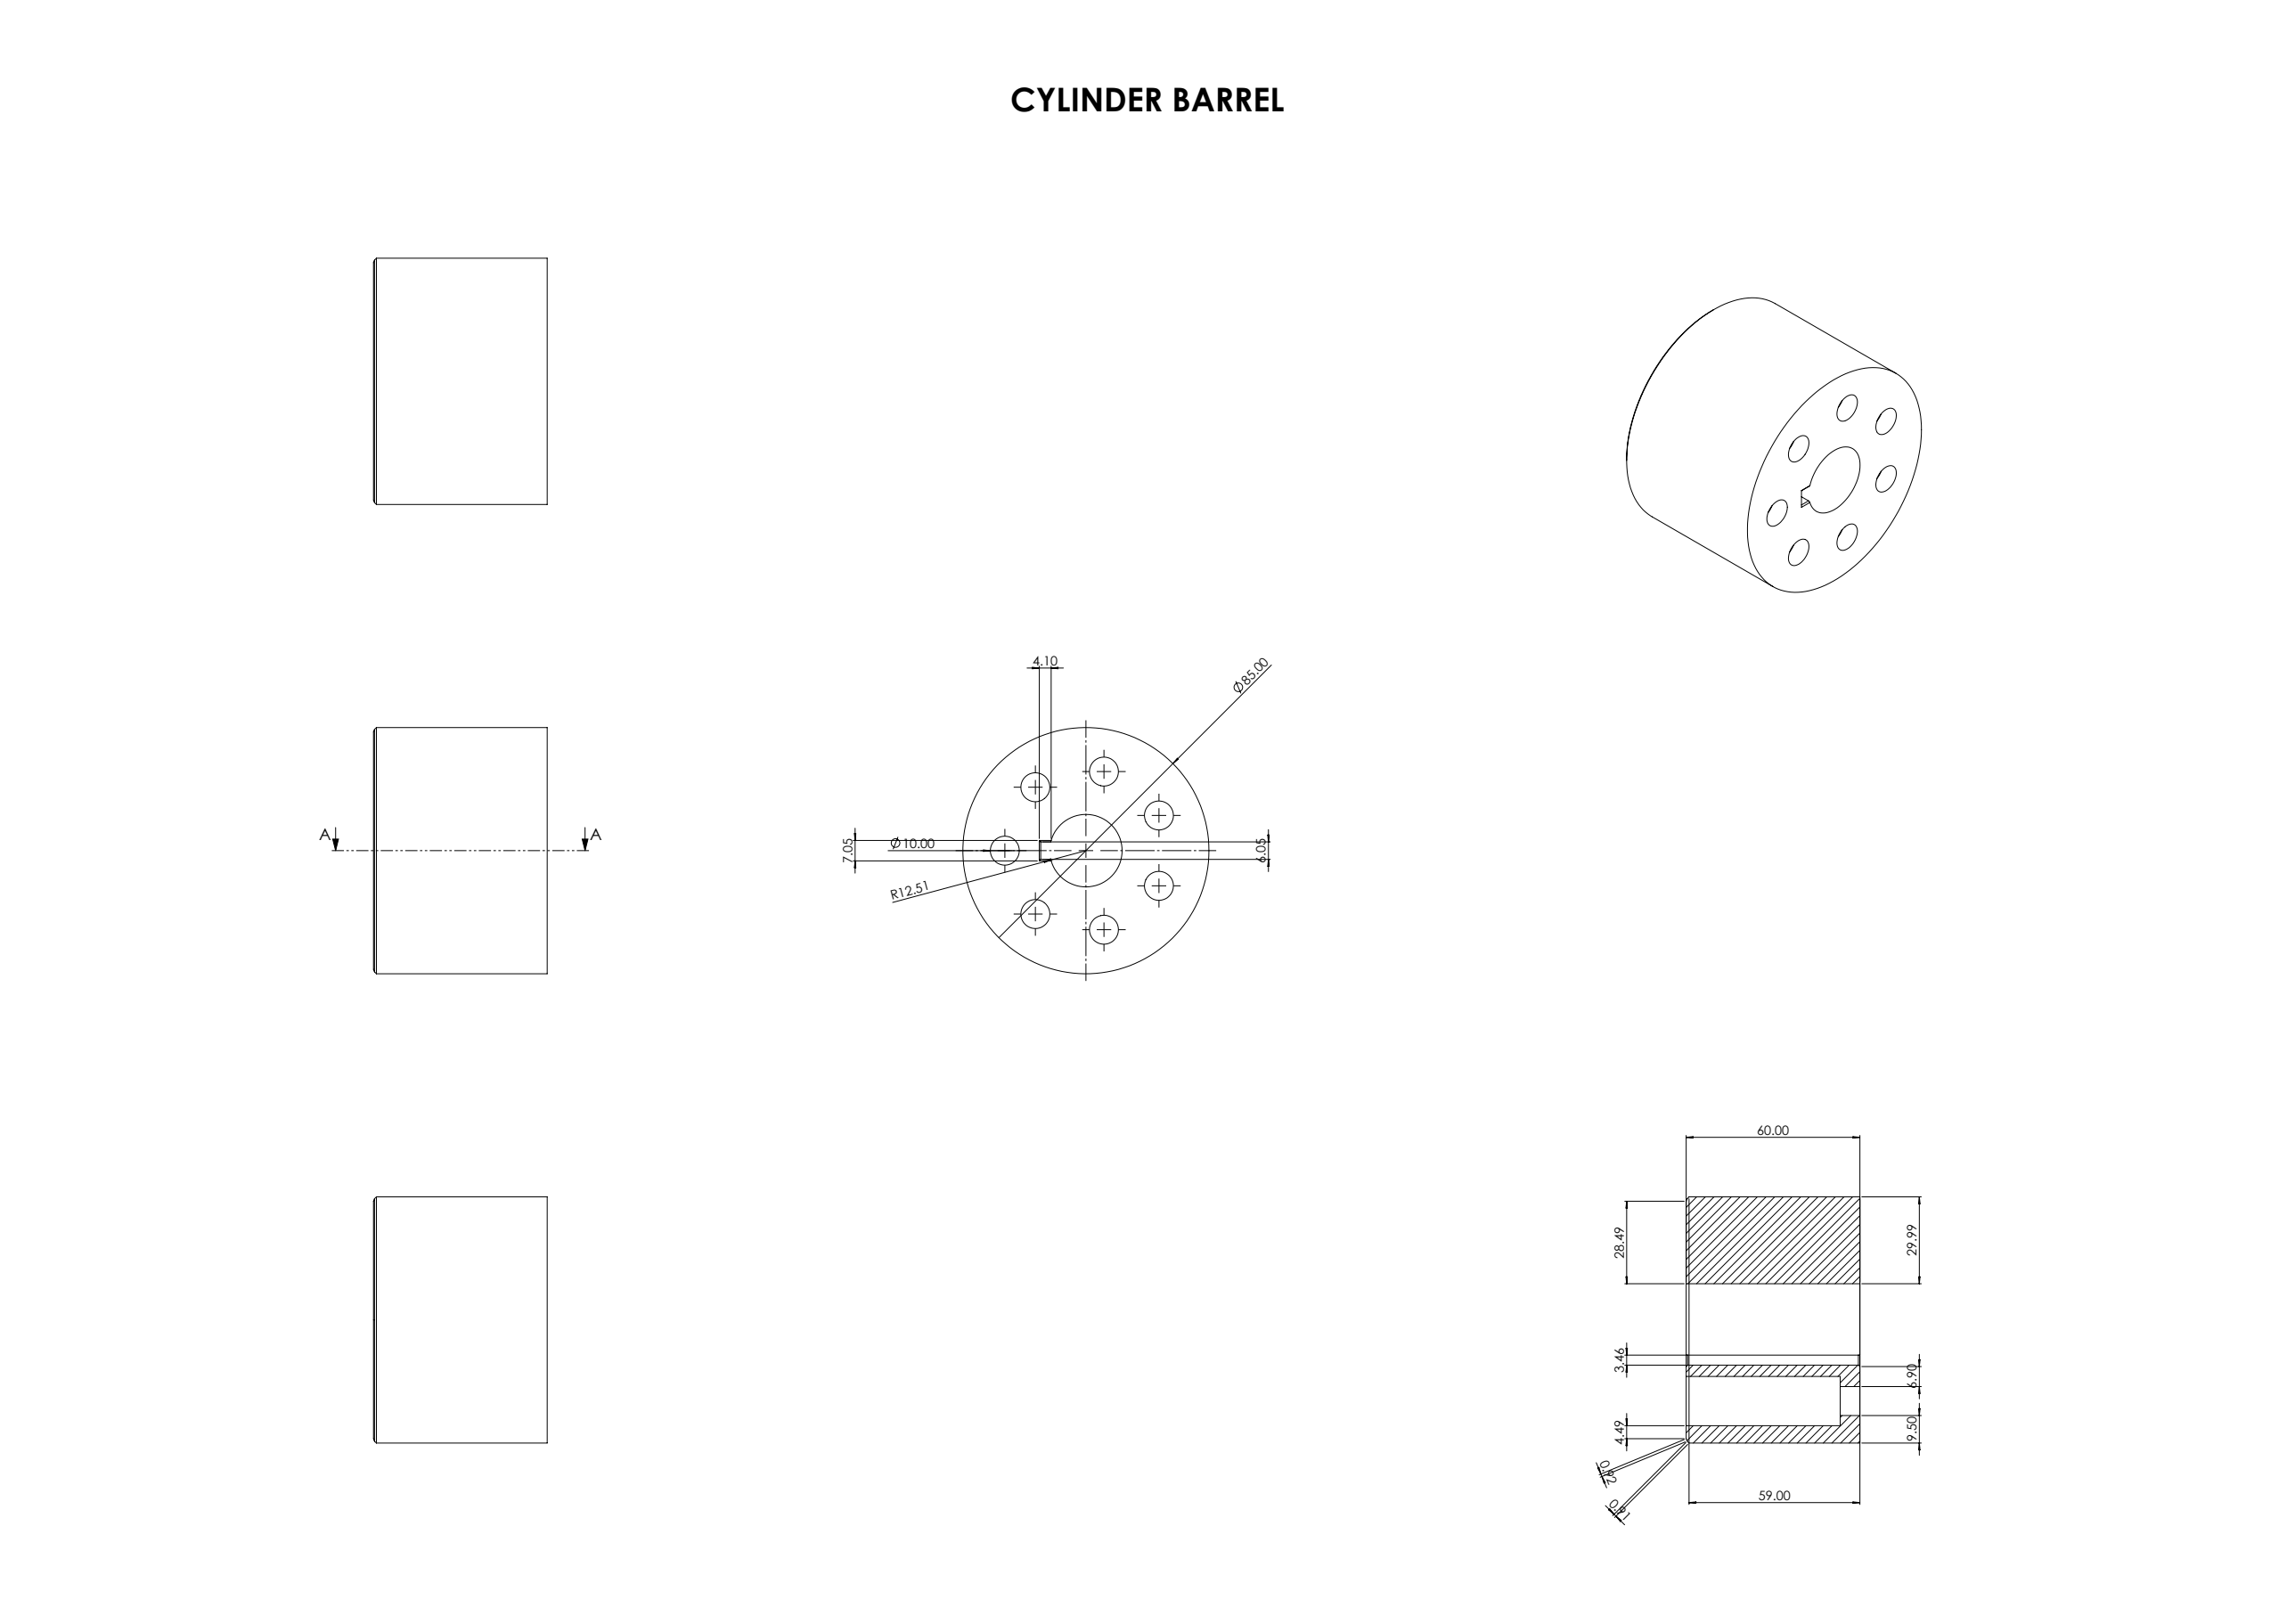
ISO-10303-21;
HEADER;
/* Generated by software containing ST-Developer
 * from STEP Tools, Inc. (www.steptools.com) 
 */

FILE_DESCRIPTION(
/* description */ (''),
/* implementation_level */ '2;1');

FILE_NAME(
/* name */ '04_Cylinder_Barrel.step',
/* time_stamp */ '2026-10-26T07:49:00-07:00',
/* author */ (''),
/* organization */ (''),
/* preprocessor_version */ 'ST-DEVELOPER v20.2',
/* originating_system */ 'Autodesk Translation Framework v15.15.0.0',
/* authorisation */ '');

FILE_SCHEMA (('AUTOMOTIVE_DESIGN { 1 0 10303 214 3 1 1 }'));
ENDSEC;

DATA;
#10=MECHANICAL_DESIGN_GEOMETRIC_PRESENTATION_REPRESENTATION('',(#180),#38507);
#150=SHAPE_REPRESENTATION_RELATIONSHIP('SRR','None',#38578,#165);
#165=ADVANCED_BREP_SHAPE_REPRESENTATION('',(#195),#38495);
#180=STYLED_ITEM('',(#38734),#195);
#195=MANIFOLD_SOLID_BREP('Body1',#15074);
#312=ELLIPSE('',#15842,17.6918116652872,12.51);
#313=ELLIPSE('',#15844,17.6918116652872,12.51);
#314=ELLIPSE('',#15849,17.6918116652872,12.51);
#315=ELLIPSE('',#15851,17.6918116652879,12.51);
#457=FACE_BOUND('',#2851,.T.);
#458=FACE_BOUND('',#2852,.T.);
#459=FACE_BOUND('',#2853,.T.);
#460=FACE_BOUND('',#2854,.T.);
#461=FACE_BOUND('',#2855,.T.);
#462=FACE_BOUND('',#2856,.T.);
#463=FACE_BOUND('',#2857,.T.);
#464=FACE_BOUND('',#2858,.T.);
#465=FACE_BOUND('',#2871,.T.);
#466=FACE_BOUND('',#2872,.T.);
#467=FACE_BOUND('',#2873,.T.);
#468=FACE_BOUND('',#2874,.T.);
#469=FACE_BOUND('',#2875,.T.);
#470=FACE_BOUND('',#2876,.T.);
#471=FACE_BOUND('',#2877,.T.);
#472=FACE_BOUND('',#2878,.T.);
#473=FACE_BOUND('',#2882,.T.);
#474=FACE_BOUND('',#2886,.T.);
#475=FACE_BOUND('',#2890,.T.);
#476=FACE_BOUND('',#2894,.T.);
#477=FACE_BOUND('',#2898,.T.);
#478=FACE_BOUND('',#2902,.T.);
#479=FACE_BOUND('',#2906,.T.);
#634=PLANE('',#15830);
#635=PLANE('',#15841);
#636=PLANE('',#15843);
#637=PLANE('',#15845);
#638=PLANE('',#15846);
#639=PLANE('',#15847);
#640=PLANE('',#15852);
#641=PLANE('',#15853);
#642=PLANE('',#15854);
#643=PLANE('',#15855);
#644=PLANE('',#15856);
#645=PLANE('',#15869);
#646=PLANE('',#15874);
#647=PLANE('',#15879);
#648=PLANE('',#15884);
#649=PLANE('',#15889);
#650=PLANE('',#15894);
#651=PLANE('',#15899);
#1467=CYLINDRICAL_SURFACE('',#15848,12.51);
#1468=CYLINDRICAL_SURFACE('',#15865,5.);
#1469=CYLINDRICAL_SURFACE('',#15867,8.51);
#1470=CYLINDRICAL_SURFACE('',#15870,5.);
#1471=CYLINDRICAL_SURFACE('',#15872,8.51);
#1472=CYLINDRICAL_SURFACE('',#15875,5.);
#1473=CYLINDRICAL_SURFACE('',#15877,8.51);
#1474=CYLINDRICAL_SURFACE('',#15880,5.);
#1475=CYLINDRICAL_SURFACE('',#15882,8.51);
#1476=CYLINDRICAL_SURFACE('',#15885,5.);
#1477=CYLINDRICAL_SURFACE('',#15887,8.51);
#1478=CYLINDRICAL_SURFACE('',#15890,5.);
#1479=CYLINDRICAL_SURFACE('',#15892,8.51);
#1480=CYLINDRICAL_SURFACE('',#15895,5.);
#1481=CYLINDRICAL_SURFACE('',#15897,8.51);
#1482=CYLINDRICAL_SURFACE('',#15900,42.5);
#1922=FACE_OUTER_BOUND('',#2849,.T.);
#1923=FACE_OUTER_BOUND('',#2850,.T.);
#1924=FACE_OUTER_BOUND('',#2859,.T.);
#1925=FACE_OUTER_BOUND('',#2860,.T.);
#1926=FACE_OUTER_BOUND('',#2861,.T.);
#1927=FACE_OUTER_BOUND('',#2862,.T.);
#1928=FACE_OUTER_BOUND('',#2863,.T.);
#1929=FACE_OUTER_BOUND('',#2864,.T.);
#1930=FACE_OUTER_BOUND('',#2865,.T.);
#1931=FACE_OUTER_BOUND('',#2866,.T.);
#1932=FACE_OUTER_BOUND('',#2867,.T.);
#1933=FACE_OUTER_BOUND('',#2868,.T.);
#1934=FACE_OUTER_BOUND('',#2869,.T.);
#1935=FACE_OUTER_BOUND('',#2870,.T.);
#1936=FACE_OUTER_BOUND('',#2879,.T.);
#1937=FACE_OUTER_BOUND('',#2880,.T.);
#1938=FACE_OUTER_BOUND('',#2881,.T.);
#1939=FACE_OUTER_BOUND('',#2883,.T.);
#1940=FACE_OUTER_BOUND('',#2884,.T.);
#1941=FACE_OUTER_BOUND('',#2885,.T.);
#1942=FACE_OUTER_BOUND('',#2887,.T.);
#1943=FACE_OUTER_BOUND('',#2888,.T.);
#1944=FACE_OUTER_BOUND('',#2889,.T.);
#1945=FACE_OUTER_BOUND('',#2891,.T.);
#1946=FACE_OUTER_BOUND('',#2892,.T.);
#1947=FACE_OUTER_BOUND('',#2893,.T.);
#1948=FACE_OUTER_BOUND('',#2895,.T.);
#1949=FACE_OUTER_BOUND('',#2896,.T.);
#1950=FACE_OUTER_BOUND('',#2897,.T.);
#1951=FACE_OUTER_BOUND('',#2899,.T.);
#1952=FACE_OUTER_BOUND('',#2900,.T.);
#1953=FACE_OUTER_BOUND('',#2901,.T.);
#1954=FACE_OUTER_BOUND('',#2903,.T.);
#1955=FACE_OUTER_BOUND('',#2904,.T.);
#1956=FACE_OUTER_BOUND('',#2905,.T.);
#1957=FACE_OUTER_BOUND('',#2907,.T.);
#2849=EDGE_LOOP('',(#11237,#11238,#11239,#11240,#11241));
#2850=EDGE_LOOP('',(#11242));
#2851=EDGE_LOOP('',(#11243));
#2852=EDGE_LOOP('',(#11244));
#2853=EDGE_LOOP('',(#11245));
#2854=EDGE_LOOP('',(#11246));
#2855=EDGE_LOOP('',(#11247));
#2856=EDGE_LOOP('',(#11248));
#2857=EDGE_LOOP('',(#11249));
#2858=EDGE_LOOP('',(#11250,#11251,#11252,#11253));
#2859=EDGE_LOOP('',(#11254,#11255,#11256,#11257,#11258));
#2860=EDGE_LOOP('',(#11259,#11260,#11261,#11262));
#2861=EDGE_LOOP('',(#11263,#11264,#11265,#11266));
#2862=EDGE_LOOP('',(#11267,#11268,#11269,#11270));
#2863=EDGE_LOOP('',(#11271,#11272,#11273,#11274));
#2864=EDGE_LOOP('',(#11275,#11276,#11277,#11278));
#2865=EDGE_LOOP('',(#11279,#11280,#11281,#11282,#11283,#11284,#11285,#11286));
#2866=EDGE_LOOP('',(#11287,#11288,#11289,#11290));
#2867=EDGE_LOOP('',(#11291,#11292,#11293,#11294));
#2868=EDGE_LOOP('',(#11295,#11296,#11297,#11298));
#2869=EDGE_LOOP('',(#11299,#11300,#11301,#11302));
#2870=EDGE_LOOP('',(#11303));
#2871=EDGE_LOOP('',(#11304,#11305,#11306,#11307));
#2872=EDGE_LOOP('',(#11308));
#2873=EDGE_LOOP('',(#11309));
#2874=EDGE_LOOP('',(#11310));
#2875=EDGE_LOOP('',(#11311));
#2876=EDGE_LOOP('',(#11312));
#2877=EDGE_LOOP('',(#11313));
#2878=EDGE_LOOP('',(#11314));
#2879=EDGE_LOOP('',(#11315,#11316,#11317,#11318));
#2880=EDGE_LOOP('',(#11319,#11320,#11321,#11322));
#2881=EDGE_LOOP('',(#11323));
#2882=EDGE_LOOP('',(#11324));
#2883=EDGE_LOOP('',(#11325,#11326,#11327,#11328));
#2884=EDGE_LOOP('',(#11329,#11330,#11331,#11332));
#2885=EDGE_LOOP('',(#11333));
#2886=EDGE_LOOP('',(#11334));
#2887=EDGE_LOOP('',(#11335,#11336,#11337,#11338));
#2888=EDGE_LOOP('',(#11339,#11340,#11341,#11342));
#2889=EDGE_LOOP('',(#11343));
#2890=EDGE_LOOP('',(#11344));
#2891=EDGE_LOOP('',(#11345,#11346,#11347,#11348));
#2892=EDGE_LOOP('',(#11349,#11350,#11351,#11352));
#2893=EDGE_LOOP('',(#11353));
#2894=EDGE_LOOP('',(#11354));
#2895=EDGE_LOOP('',(#11355,#11356,#11357,#11358));
#2896=EDGE_LOOP('',(#11359,#11360,#11361,#11362));
#2897=EDGE_LOOP('',(#11363));
#2898=EDGE_LOOP('',(#11364));
#2899=EDGE_LOOP('',(#11365,#11366,#11367,#11368));
#2900=EDGE_LOOP('',(#11369,#11370,#11371,#11372));
#2901=EDGE_LOOP('',(#11373));
#2902=EDGE_LOOP('',(#11374));
#2903=EDGE_LOOP('',(#11375,#11376,#11377,#11378));
#2904=EDGE_LOOP('',(#11379,#11380,#11381,#11382));
#2905=EDGE_LOOP('',(#11383));
#2906=EDGE_LOOP('',(#11384));
#2907=EDGE_LOOP('',(#11385,#11386,#11387,#11388));
#3783=LINE('',#25475,#4852);
#3784=LINE('',#25494,#4853);
#3785=LINE('',#25498,#4854);
#3786=LINE('',#25499,#4855);
#3787=LINE('',#25503,#4856);
#3788=LINE('',#25507,#4857);
#3789=LINE('',#25509,#4858);
#3790=LINE('',#25514,#4859);
#3791=LINE('',#25515,#4860);
#3792=LINE('',#25517,#4861);
#3793=LINE('',#25520,#4862);
#3794=LINE('',#25522,#4863);
#3795=LINE('',#25523,#4864);
#3796=LINE('',#25526,#4865);
#3797=LINE('',#25527,#4866);
#3798=LINE('',#25535,#4867);
#3799=LINE('',#25537,#4868);
#3800=LINE('',#25540,#4869);
#3801=LINE('',#25541,#4870);
#3802=LINE('',#25544,#4871);
#3803=LINE('',#25545,#4872);
#3804=LINE('',#25547,#4873);
#3805=LINE('',#25567,#4874);
#3806=LINE('',#25571,#4875);
#3807=LINE('',#25576,#4876);
#3808=LINE('',#25580,#4877);
#3809=LINE('',#25585,#4878);
#3810=LINE('',#25589,#4879);
#3811=LINE('',#25594,#4880);
#3812=LINE('',#25598,#4881);
#3813=LINE('',#25603,#4882);
#3814=LINE('',#25607,#4883);
#3815=LINE('',#25612,#4884);
#3816=LINE('',#25616,#4885);
#3817=LINE('',#25621,#4886);
#3818=LINE('',#25625,#4887);
#3819=LINE('',#25629,#4888);
#4852=VECTOR('',#18180,41.4267766952966);
#4853=VECTOR('',#18199,10.);
#4854=VECTOR('',#18202,10.);
#4855=VECTOR('',#18203,10.);
#4856=VECTOR('',#18208,42.);
#4857=VECTOR('',#18211,10.);
#4858=VECTOR('',#18214,10.);
#4859=VECTOR('',#18219,10.);
#4860=VECTOR('',#18220,10.);
#4861=VECTOR('',#18223,10.);
#4862=VECTOR('',#18226,10.);
#4863=VECTOR('',#18227,10.);
#4864=VECTOR('',#18228,10.);
#4865=VECTOR('',#18231,10.);
#4866=VECTOR('',#18232,10.);
#4867=VECTOR('',#18241,10.);
#4868=VECTOR('',#18244,10.);
#4869=VECTOR('',#18247,10.);
#4870=VECTOR('',#18248,10.);
#4871=VECTOR('',#18251,10.);
#4872=VECTOR('',#18252,10.);
#4873=VECTOR('',#18255,10.);
#4874=VECTOR('',#18276,5.);
#4875=VECTOR('',#18281,8.51);
#4876=VECTOR('',#18288,5.);
#4877=VECTOR('',#18293,8.51);
#4878=VECTOR('',#18300,5.);
#4879=VECTOR('',#18305,8.51);
#4880=VECTOR('',#18312,5.);
#4881=VECTOR('',#18317,8.51);
#4882=VECTOR('',#18324,5.);
#4883=VECTOR('',#18329,8.51);
#4884=VECTOR('',#18336,5.);
#4885=VECTOR('',#18341,8.51);
#4886=VECTOR('',#18348,5.);
#4887=VECTOR('',#18353,8.51);
#4888=VECTOR('',#18360,42.5);
#5960=CIRCLE('',#15827,41.8535533905933);
#5961=CIRCLE('',#15828,41.8535533905933);
#5962=CIRCLE('',#15829,41.);
#5963=CIRCLE('',#15831,8.51);
#5964=CIRCLE('',#15832,8.51);
#5965=CIRCLE('',#15833,8.51);
#5966=CIRCLE('',#15834,8.51);
#5967=CIRCLE('',#15835,8.51);
#5968=CIRCLE('',#15836,8.51);
#5969=CIRCLE('',#15837,8.51);
#5970=CIRCLE('',#15838,12.51);
#5971=CIRCLE('',#15840,42.5);
#5972=CIRCLE('',#15850,12.51);
#5973=CIRCLE('',#15857,42.5);
#5974=CIRCLE('',#15858,5.);
#5975=CIRCLE('',#15859,5.);
#5976=CIRCLE('',#15860,5.);
#5977=CIRCLE('',#15861,5.);
#5978=CIRCLE('',#15862,5.);
#5979=CIRCLE('',#15863,5.);
#5980=CIRCLE('',#15864,5.);
#5981=CIRCLE('',#15866,5.);
#5982=CIRCLE('',#15868,8.51);
#5983=CIRCLE('',#15871,5.);
#5984=CIRCLE('',#15873,8.51);
#5985=CIRCLE('',#15876,5.);
#5986=CIRCLE('',#15878,8.51);
#5987=CIRCLE('',#15881,5.);
#5988=CIRCLE('',#15883,8.51);
#5989=CIRCLE('',#15886,5.);
#5990=CIRCLE('',#15888,8.51);
#5991=CIRCLE('',#15891,5.);
#5992=CIRCLE('',#15893,8.51);
#5993=CIRCLE('',#15896,5.);
#5994=CIRCLE('',#15898,8.51);
#6707=VERTEX_POINT('',#25470);
#6708=VERTEX_POINT('',#25471);
#6709=VERTEX_POINT('',#25474);
#6710=VERTEX_POINT('',#25478);
#6711=VERTEX_POINT('',#25480);
#6712=VERTEX_POINT('',#25482);
#6713=VERTEX_POINT('',#25484);
#6714=VERTEX_POINT('',#25486);
#6715=VERTEX_POINT('',#25488);
#6716=VERTEX_POINT('',#25490);
#6717=VERTEX_POINT('',#25492);
#6718=VERTEX_POINT('',#25493);
#6719=VERTEX_POINT('',#25495);
#6720=VERTEX_POINT('',#25497);
#6721=VERTEX_POINT('',#25501);
#6722=VERTEX_POINT('',#25505);
#6723=VERTEX_POINT('',#25506);
#6724=VERTEX_POINT('',#25511);
#6725=VERTEX_POINT('',#25513);
#6726=VERTEX_POINT('',#25519);
#6727=VERTEX_POINT('',#25521);
#6728=VERTEX_POINT('',#25525);
#6729=VERTEX_POINT('',#25529);
#6730=VERTEX_POINT('',#25531);
#6731=VERTEX_POINT('',#25533);
#6732=VERTEX_POINT('',#25539);
#6733=VERTEX_POINT('',#25543);
#6734=VERTEX_POINT('',#25549);
#6735=VERTEX_POINT('',#25551);
#6736=VERTEX_POINT('',#25553);
#6737=VERTEX_POINT('',#25555);
#6738=VERTEX_POINT('',#25557);
#6739=VERTEX_POINT('',#25559);
#6740=VERTEX_POINT('',#25561);
#6741=VERTEX_POINT('',#25563);
#6742=VERTEX_POINT('',#25566);
#6743=VERTEX_POINT('',#25570);
#6744=VERTEX_POINT('',#25575);
#6745=VERTEX_POINT('',#25579);
#6746=VERTEX_POINT('',#25584);
#6747=VERTEX_POINT('',#25588);
#6748=VERTEX_POINT('',#25593);
#6749=VERTEX_POINT('',#25597);
#6750=VERTEX_POINT('',#25602);
#6751=VERTEX_POINT('',#25606);
#6752=VERTEX_POINT('',#25611);
#6753=VERTEX_POINT('',#25615);
#6754=VERTEX_POINT('',#25620);
#6755=VERTEX_POINT('',#25624);
#8367=EDGE_CURVE('',#6707,#6708,#5960,.T.);
#8368=EDGE_CURVE('',#6708,#6707,#5961,.T.);
#8369=EDGE_CURVE('',#6707,#6709,#3783,.T.);
#8370=EDGE_CURVE('',#6709,#6709,#5962,.T.);
#8371=EDGE_CURVE('',#6710,#6710,#5963,.T.);
#8372=EDGE_CURVE('',#6711,#6711,#5964,.T.);
#8373=EDGE_CURVE('',#6712,#6712,#5965,.T.);
#8374=EDGE_CURVE('',#6713,#6713,#5966,.T.);
#8375=EDGE_CURVE('',#6714,#6714,#5967,.T.);
#8376=EDGE_CURVE('',#6715,#6715,#5968,.T.);
#8377=EDGE_CURVE('',#6716,#6716,#5969,.T.);
#8378=EDGE_CURVE('',#6717,#6718,#3784,.T.);
#8379=EDGE_CURVE('',#6717,#6719,#5970,.T.);
#8380=EDGE_CURVE('',#6720,#6719,#3785,.T.);
#8381=EDGE_CURVE('',#6718,#6720,#3786,.T.);
#8382=EDGE_CURVE('',#6721,#6721,#5971,.T.);
#8383=EDGE_CURVE('',#6721,#6708,#3787,.T.);
#8384=EDGE_CURVE('',#6722,#6723,#3788,.T.);
#8385=EDGE_CURVE('',#6723,#6717,#312,.T.);
#8386=EDGE_CURVE('',#6718,#6722,#3789,.T.);
#8387=EDGE_CURVE('',#6719,#6724,#313,.T.);
#8388=EDGE_CURVE('',#6724,#6725,#3790,.T.);
#8389=EDGE_CURVE('',#6725,#6720,#3791,.T.);
#8390=EDGE_CURVE('',#6725,#6722,#3792,.T.);
#8391=EDGE_CURVE('',#6722,#6726,#3793,.T.);
#8392=EDGE_CURVE('',#6727,#6726,#3794,.T.);
#8393=EDGE_CURVE('',#6723,#6727,#3795,.T.);
#8394=EDGE_CURVE('',#6728,#6725,#3796,.T.);
#8395=EDGE_CURVE('',#6726,#6728,#3797,.T.);
#8396=EDGE_CURVE('',#6729,#6727,#314,.T.);
#8397=EDGE_CURVE('',#6729,#6730,#5972,.T.);
#8398=EDGE_CURVE('',#6731,#6730,#315,.T.);
#8399=EDGE_CURVE('',#6731,#6724,#3798,.T.);
#8400=EDGE_CURVE('',#6728,#6731,#3799,.T.);
#8401=EDGE_CURVE('',#6732,#6729,#3800,.T.);
#8402=EDGE_CURVE('',#6726,#6732,#3801,.T.);
#8403=EDGE_CURVE('',#6730,#6733,#3802,.T.);
#8404=EDGE_CURVE('',#6733,#6728,#3803,.T.);
#8405=EDGE_CURVE('',#6733,#6732,#3804,.T.);
#8406=EDGE_CURVE('',#6734,#6734,#5973,.T.);
#8407=EDGE_CURVE('',#6735,#6735,#5974,.T.);
#8408=EDGE_CURVE('',#6736,#6736,#5975,.T.);
#8409=EDGE_CURVE('',#6737,#6737,#5976,.T.);
#8410=EDGE_CURVE('',#6738,#6738,#5977,.T.);
#8411=EDGE_CURVE('',#6739,#6739,#5978,.T.);
#8412=EDGE_CURVE('',#6740,#6740,#5979,.T.);
#8413=EDGE_CURVE('',#6741,#6741,#5980,.T.);
#8414=EDGE_CURVE('',#6741,#6742,#3805,.T.);
#8415=EDGE_CURVE('',#6742,#6742,#5981,.T.);
#8416=EDGE_CURVE('',#6716,#6743,#3806,.T.);
#8417=EDGE_CURVE('',#6743,#6743,#5982,.T.);
#8418=EDGE_CURVE('',#6740,#6744,#3807,.T.);
#8419=EDGE_CURVE('',#6744,#6744,#5983,.T.);
#8420=EDGE_CURVE('',#6715,#6745,#3808,.T.);
#8421=EDGE_CURVE('',#6745,#6745,#5984,.T.);
#8422=EDGE_CURVE('',#6739,#6746,#3809,.T.);
#8423=EDGE_CURVE('',#6746,#6746,#5985,.T.);
#8424=EDGE_CURVE('',#6714,#6747,#3810,.T.);
#8425=EDGE_CURVE('',#6747,#6747,#5986,.T.);
#8426=EDGE_CURVE('',#6738,#6748,#3811,.T.);
#8427=EDGE_CURVE('',#6748,#6748,#5987,.T.);
#8428=EDGE_CURVE('',#6713,#6749,#3812,.T.);
#8429=EDGE_CURVE('',#6749,#6749,#5988,.T.);
#8430=EDGE_CURVE('',#6737,#6750,#3813,.T.);
#8431=EDGE_CURVE('',#6750,#6750,#5989,.T.);
#8432=EDGE_CURVE('',#6712,#6751,#3814,.T.);
#8433=EDGE_CURVE('',#6751,#6751,#5990,.T.);
#8434=EDGE_CURVE('',#6736,#6752,#3815,.T.);
#8435=EDGE_CURVE('',#6752,#6752,#5991,.T.);
#8436=EDGE_CURVE('',#6711,#6753,#3816,.T.);
#8437=EDGE_CURVE('',#6753,#6753,#5992,.T.);
#8438=EDGE_CURVE('',#6735,#6754,#3817,.T.);
#8439=EDGE_CURVE('',#6754,#6754,#5993,.T.);
#8440=EDGE_CURVE('',#6710,#6755,#3818,.T.);
#8441=EDGE_CURVE('',#6755,#6755,#5994,.T.);
#8442=EDGE_CURVE('',#6734,#6721,#3819,.T.);
#11237=ORIENTED_EDGE('',*,*,#8367,.T.);
#11238=ORIENTED_EDGE('',*,*,#8368,.T.);
#11239=ORIENTED_EDGE('',*,*,#8369,.T.);
#11240=ORIENTED_EDGE('',*,*,#8370,.T.);
#11241=ORIENTED_EDGE('',*,*,#8369,.F.);
#11242=ORIENTED_EDGE('',*,*,#8370,.F.);
#11243=ORIENTED_EDGE('',*,*,#8371,.T.);
#11244=ORIENTED_EDGE('',*,*,#8372,.T.);
#11245=ORIENTED_EDGE('',*,*,#8373,.T.);
#11246=ORIENTED_EDGE('',*,*,#8374,.T.);
#11247=ORIENTED_EDGE('',*,*,#8375,.T.);
#11248=ORIENTED_EDGE('',*,*,#8376,.T.);
#11249=ORIENTED_EDGE('',*,*,#8377,.T.);
#11250=ORIENTED_EDGE('',*,*,#8378,.F.);
#11251=ORIENTED_EDGE('',*,*,#8379,.T.);
#11252=ORIENTED_EDGE('',*,*,#8380,.F.);
#11253=ORIENTED_EDGE('',*,*,#8381,.F.);
#11254=ORIENTED_EDGE('',*,*,#8382,.F.);
#11255=ORIENTED_EDGE('',*,*,#8383,.T.);
#11256=ORIENTED_EDGE('',*,*,#8367,.F.);
#11257=ORIENTED_EDGE('',*,*,#8368,.F.);
#11258=ORIENTED_EDGE('',*,*,#8383,.F.);
#11259=ORIENTED_EDGE('',*,*,#8384,.T.);
#11260=ORIENTED_EDGE('',*,*,#8385,.T.);
#11261=ORIENTED_EDGE('',*,*,#8378,.T.);
#11262=ORIENTED_EDGE('',*,*,#8386,.T.);
#11263=ORIENTED_EDGE('',*,*,#8380,.T.);
#11264=ORIENTED_EDGE('',*,*,#8387,.T.);
#11265=ORIENTED_EDGE('',*,*,#8388,.T.);
#11266=ORIENTED_EDGE('',*,*,#8389,.T.);
#11267=ORIENTED_EDGE('',*,*,#8381,.T.);
#11268=ORIENTED_EDGE('',*,*,#8389,.F.);
#11269=ORIENTED_EDGE('',*,*,#8390,.T.);
#11270=ORIENTED_EDGE('',*,*,#8386,.F.);
#11271=ORIENTED_EDGE('',*,*,#8384,.F.);
#11272=ORIENTED_EDGE('',*,*,#8391,.T.);
#11273=ORIENTED_EDGE('',*,*,#8392,.F.);
#11274=ORIENTED_EDGE('',*,*,#8393,.F.);
#11275=ORIENTED_EDGE('',*,*,#8390,.F.);
#11276=ORIENTED_EDGE('',*,*,#8394,.F.);
#11277=ORIENTED_EDGE('',*,*,#8395,.F.);
#11278=ORIENTED_EDGE('',*,*,#8391,.F.);
#11279=ORIENTED_EDGE('',*,*,#8385,.F.);
#11280=ORIENTED_EDGE('',*,*,#8393,.T.);
#11281=ORIENTED_EDGE('',*,*,#8396,.F.);
#11282=ORIENTED_EDGE('',*,*,#8397,.T.);
#11283=ORIENTED_EDGE('',*,*,#8398,.F.);
#11284=ORIENTED_EDGE('',*,*,#8399,.T.);
#11285=ORIENTED_EDGE('',*,*,#8387,.F.);
#11286=ORIENTED_EDGE('',*,*,#8379,.F.);
#11287=ORIENTED_EDGE('',*,*,#8388,.F.);
#11288=ORIENTED_EDGE('',*,*,#8399,.F.);
#11289=ORIENTED_EDGE('',*,*,#8400,.F.);
#11290=ORIENTED_EDGE('',*,*,#8394,.T.);
#11291=ORIENTED_EDGE('',*,*,#8401,.T.);
#11292=ORIENTED_EDGE('',*,*,#8396,.T.);
#11293=ORIENTED_EDGE('',*,*,#8392,.T.);
#11294=ORIENTED_EDGE('',*,*,#8402,.T.);
#11295=ORIENTED_EDGE('',*,*,#8400,.T.);
#11296=ORIENTED_EDGE('',*,*,#8398,.T.);
#11297=ORIENTED_EDGE('',*,*,#8403,.T.);
#11298=ORIENTED_EDGE('',*,*,#8404,.T.);
#11299=ORIENTED_EDGE('',*,*,#8395,.T.);
#11300=ORIENTED_EDGE('',*,*,#8404,.F.);
#11301=ORIENTED_EDGE('',*,*,#8405,.T.);
#11302=ORIENTED_EDGE('',*,*,#8402,.F.);
#11303=ORIENTED_EDGE('',*,*,#8406,.T.);
#11304=ORIENTED_EDGE('',*,*,#8401,.F.);
#11305=ORIENTED_EDGE('',*,*,#8405,.F.);
#11306=ORIENTED_EDGE('',*,*,#8403,.F.);
#11307=ORIENTED_EDGE('',*,*,#8397,.F.);
#11308=ORIENTED_EDGE('',*,*,#8407,.T.);
#11309=ORIENTED_EDGE('',*,*,#8408,.T.);
#11310=ORIENTED_EDGE('',*,*,#8409,.T.);
#11311=ORIENTED_EDGE('',*,*,#8410,.T.);
#11312=ORIENTED_EDGE('',*,*,#8411,.T.);
#11313=ORIENTED_EDGE('',*,*,#8412,.T.);
#11314=ORIENTED_EDGE('',*,*,#8413,.T.);
#11315=ORIENTED_EDGE('',*,*,#8413,.F.);
#11316=ORIENTED_EDGE('',*,*,#8414,.T.);
#11317=ORIENTED_EDGE('',*,*,#8415,.F.);
#11318=ORIENTED_EDGE('',*,*,#8414,.F.);
#11319=ORIENTED_EDGE('',*,*,#8377,.F.);
#11320=ORIENTED_EDGE('',*,*,#8416,.T.);
#11321=ORIENTED_EDGE('',*,*,#8417,.T.);
#11322=ORIENTED_EDGE('',*,*,#8416,.F.);
#11323=ORIENTED_EDGE('',*,*,#8417,.F.);
#11324=ORIENTED_EDGE('',*,*,#8415,.T.);
#11325=ORIENTED_EDGE('',*,*,#8412,.F.);
#11326=ORIENTED_EDGE('',*,*,#8418,.T.);
#11327=ORIENTED_EDGE('',*,*,#8419,.F.);
#11328=ORIENTED_EDGE('',*,*,#8418,.F.);
#11329=ORIENTED_EDGE('',*,*,#8376,.F.);
#11330=ORIENTED_EDGE('',*,*,#8420,.T.);
#11331=ORIENTED_EDGE('',*,*,#8421,.T.);
#11332=ORIENTED_EDGE('',*,*,#8420,.F.);
#11333=ORIENTED_EDGE('',*,*,#8421,.F.);
#11334=ORIENTED_EDGE('',*,*,#8419,.T.);
#11335=ORIENTED_EDGE('',*,*,#8411,.F.);
#11336=ORIENTED_EDGE('',*,*,#8422,.T.);
#11337=ORIENTED_EDGE('',*,*,#8423,.F.);
#11338=ORIENTED_EDGE('',*,*,#8422,.F.);
#11339=ORIENTED_EDGE('',*,*,#8375,.F.);
#11340=ORIENTED_EDGE('',*,*,#8424,.T.);
#11341=ORIENTED_EDGE('',*,*,#8425,.T.);
#11342=ORIENTED_EDGE('',*,*,#8424,.F.);
#11343=ORIENTED_EDGE('',*,*,#8425,.F.);
#11344=ORIENTED_EDGE('',*,*,#8423,.T.);
#11345=ORIENTED_EDGE('',*,*,#8410,.F.);
#11346=ORIENTED_EDGE('',*,*,#8426,.T.);
#11347=ORIENTED_EDGE('',*,*,#8427,.F.);
#11348=ORIENTED_EDGE('',*,*,#8426,.F.);
#11349=ORIENTED_EDGE('',*,*,#8374,.F.);
#11350=ORIENTED_EDGE('',*,*,#8428,.T.);
#11351=ORIENTED_EDGE('',*,*,#8429,.T.);
#11352=ORIENTED_EDGE('',*,*,#8428,.F.);
#11353=ORIENTED_EDGE('',*,*,#8429,.F.);
#11354=ORIENTED_EDGE('',*,*,#8427,.T.);
#11355=ORIENTED_EDGE('',*,*,#8409,.F.);
#11356=ORIENTED_EDGE('',*,*,#8430,.T.);
#11357=ORIENTED_EDGE('',*,*,#8431,.F.);
#11358=ORIENTED_EDGE('',*,*,#8430,.F.);
#11359=ORIENTED_EDGE('',*,*,#8373,.F.);
#11360=ORIENTED_EDGE('',*,*,#8432,.T.);
#11361=ORIENTED_EDGE('',*,*,#8433,.T.);
#11362=ORIENTED_EDGE('',*,*,#8432,.F.);
#11363=ORIENTED_EDGE('',*,*,#8433,.F.);
#11364=ORIENTED_EDGE('',*,*,#8431,.T.);
#11365=ORIENTED_EDGE('',*,*,#8408,.F.);
#11366=ORIENTED_EDGE('',*,*,#8434,.T.);
#11367=ORIENTED_EDGE('',*,*,#8435,.F.);
#11368=ORIENTED_EDGE('',*,*,#8434,.F.);
#11369=ORIENTED_EDGE('',*,*,#8372,.F.);
#11370=ORIENTED_EDGE('',*,*,#8436,.T.);
#11371=ORIENTED_EDGE('',*,*,#8437,.T.);
#11372=ORIENTED_EDGE('',*,*,#8436,.F.);
#11373=ORIENTED_EDGE('',*,*,#8437,.F.);
#11374=ORIENTED_EDGE('',*,*,#8435,.T.);
#11375=ORIENTED_EDGE('',*,*,#8407,.F.);
#11376=ORIENTED_EDGE('',*,*,#8438,.T.);
#11377=ORIENTED_EDGE('',*,*,#8439,.F.);
#11378=ORIENTED_EDGE('',*,*,#8438,.F.);
#11379=ORIENTED_EDGE('',*,*,#8371,.F.);
#11380=ORIENTED_EDGE('',*,*,#8440,.T.);
#11381=ORIENTED_EDGE('',*,*,#8441,.T.);
#11382=ORIENTED_EDGE('',*,*,#8440,.F.);
#11383=ORIENTED_EDGE('',*,*,#8441,.F.);
#11384=ORIENTED_EDGE('',*,*,#8439,.T.);
#11385=ORIENTED_EDGE('',*,*,#8406,.F.);
#11386=ORIENTED_EDGE('',*,*,#8442,.T.);
#11387=ORIENTED_EDGE('',*,*,#8382,.T.);
#11388=ORIENTED_EDGE('',*,*,#8442,.F.);
#14133=CONICAL_SURFACE('',#15826,41.4267766952966,1.17809724509617);
#14134=CONICAL_SURFACE('',#15839,42.,0.785398163397448);
#14489=ADVANCED_FACE('',(#1922),#14133,.T.);
#14490=ADVANCED_FACE('',(#1923,#457,#458,#459,#460,#461,#462,#463,#464),
#634,.T.);
#14491=ADVANCED_FACE('',(#1924),#14134,.T.);
#14492=ADVANCED_FACE('',(#1925),#635,.T.);
#14493=ADVANCED_FACE('',(#1926),#636,.T.);
#14494=ADVANCED_FACE('',(#1927),#637,.T.);
#14495=ADVANCED_FACE('',(#1928),#638,.F.);
#14496=ADVANCED_FACE('',(#1929),#639,.F.);
#14497=ADVANCED_FACE('',(#1930),#1467,.F.);
#14498=ADVANCED_FACE('',(#1931),#640,.F.);
#14499=ADVANCED_FACE('',(#1932),#641,.T.);
#14500=ADVANCED_FACE('',(#1933),#642,.T.);
#14501=ADVANCED_FACE('',(#1934),#643,.T.);
#14502=ADVANCED_FACE('',(#1935,#465,#466,#467,#468,#469,#470,#471,#472),
#644,.T.);
#14503=ADVANCED_FACE('',(#1936),#1468,.F.);
#14504=ADVANCED_FACE('',(#1937),#1469,.F.);
#14505=ADVANCED_FACE('',(#1938,#473),#645,.F.);
#14506=ADVANCED_FACE('',(#1939),#1470,.F.);
#14507=ADVANCED_FACE('',(#1940),#1471,.F.);
#14508=ADVANCED_FACE('',(#1941,#474),#646,.F.);
#14509=ADVANCED_FACE('',(#1942),#1472,.F.);
#14510=ADVANCED_FACE('',(#1943),#1473,.F.);
#14511=ADVANCED_FACE('',(#1944,#475),#647,.F.);
#14512=ADVANCED_FACE('',(#1945),#1474,.F.);
#14513=ADVANCED_FACE('',(#1946),#1475,.F.);
#14514=ADVANCED_FACE('',(#1947,#476),#648,.F.);
#14515=ADVANCED_FACE('',(#1948),#1476,.F.);
#14516=ADVANCED_FACE('',(#1949),#1477,.F.);
#14517=ADVANCED_FACE('',(#1950,#477),#649,.F.);
#14518=ADVANCED_FACE('',(#1951),#1478,.F.);
#14519=ADVANCED_FACE('',(#1952),#1479,.F.);
#14520=ADVANCED_FACE('',(#1953,#478),#650,.F.);
#14521=ADVANCED_FACE('',(#1954),#1480,.F.);
#14522=ADVANCED_FACE('',(#1955),#1481,.F.);
#14523=ADVANCED_FACE('',(#1956,#479),#651,.F.);
#14524=ADVANCED_FACE('',(#1957),#1482,.T.);
#15074=CLOSED_SHELL('',(#14489,#14490,#14491,#14492,#14493,#14494,#14495,
#14496,#14497,#14498,#14499,#14500,#14501,#14502,#14503,#14504,#14505,#14506,
#14507,#14508,#14509,#14510,#14511,#14512,#14513,#14514,#14515,#14516,#14517,
#14518,#14519,#14520,#14521,#14522,#14523,#14524));
#15825=AXIS2_PLACEMENT_3D('',#25468,#18172,#18173);
#15826=AXIS2_PLACEMENT_3D('',#25469,#18174,#18175);
#15827=AXIS2_PLACEMENT_3D('',#25472,#18176,#18177);
#15828=AXIS2_PLACEMENT_3D('',#25473,#18178,#18179);
#15829=AXIS2_PLACEMENT_3D('',#25476,#18181,#18182);
#15830=AXIS2_PLACEMENT_3D('',#25477,#18183,#18184);
#15831=AXIS2_PLACEMENT_3D('',#25479,#18185,#18186);
#15832=AXIS2_PLACEMENT_3D('',#25481,#18187,#18188);
#15833=AXIS2_PLACEMENT_3D('',#25483,#18189,#18190);
#15834=AXIS2_PLACEMENT_3D('',#25485,#18191,#18192);
#15835=AXIS2_PLACEMENT_3D('',#25487,#18193,#18194);
#15836=AXIS2_PLACEMENT_3D('',#25489,#18195,#18196);
#15837=AXIS2_PLACEMENT_3D('',#25491,#18197,#18198);
#15838=AXIS2_PLACEMENT_3D('',#25496,#18200,#18201);
#15839=AXIS2_PLACEMENT_3D('',#25500,#18204,#18205);
#15840=AXIS2_PLACEMENT_3D('',#25502,#18206,#18207);
#15841=AXIS2_PLACEMENT_3D('',#25504,#18209,#18210);
#15842=AXIS2_PLACEMENT_3D('',#25508,#18212,#18213);
#15843=AXIS2_PLACEMENT_3D('',#25510,#18215,#18216);
#15844=AXIS2_PLACEMENT_3D('',#25512,#18217,#18218);
#15845=AXIS2_PLACEMENT_3D('',#25516,#18221,#18222);
#15846=AXIS2_PLACEMENT_3D('',#25518,#18224,#18225);
#15847=AXIS2_PLACEMENT_3D('',#25524,#18229,#18230);
#15848=AXIS2_PLACEMENT_3D('',#25528,#18233,#18234);
#15849=AXIS2_PLACEMENT_3D('',#25530,#18235,#18236);
#15850=AXIS2_PLACEMENT_3D('',#25532,#18237,#18238);
#15851=AXIS2_PLACEMENT_3D('',#25534,#18239,#18240);
#15852=AXIS2_PLACEMENT_3D('',#25536,#18242,#18243);
#15853=AXIS2_PLACEMENT_3D('',#25538,#18245,#18246);
#15854=AXIS2_PLACEMENT_3D('',#25542,#18249,#18250);
#15855=AXIS2_PLACEMENT_3D('',#25546,#18253,#18254);
#15856=AXIS2_PLACEMENT_3D('',#25548,#18256,#18257);
#15857=AXIS2_PLACEMENT_3D('',#25550,#18258,#18259);
#15858=AXIS2_PLACEMENT_3D('',#25552,#18260,#18261);
#15859=AXIS2_PLACEMENT_3D('',#25554,#18262,#18263);
#15860=AXIS2_PLACEMENT_3D('',#25556,#18264,#18265);
#15861=AXIS2_PLACEMENT_3D('',#25558,#18266,#18267);
#15862=AXIS2_PLACEMENT_3D('',#25560,#18268,#18269);
#15863=AXIS2_PLACEMENT_3D('',#25562,#18270,#18271);
#15864=AXIS2_PLACEMENT_3D('',#25564,#18272,#18273);
#15865=AXIS2_PLACEMENT_3D('',#25565,#18274,#18275);
#15866=AXIS2_PLACEMENT_3D('',#25568,#18277,#18278);
#15867=AXIS2_PLACEMENT_3D('',#25569,#18279,#18280);
#15868=AXIS2_PLACEMENT_3D('',#25572,#18282,#18283);
#15869=AXIS2_PLACEMENT_3D('',#25573,#18284,#18285);
#15870=AXIS2_PLACEMENT_3D('',#25574,#18286,#18287);
#15871=AXIS2_PLACEMENT_3D('',#25577,#18289,#18290);
#15872=AXIS2_PLACEMENT_3D('',#25578,#18291,#18292);
#15873=AXIS2_PLACEMENT_3D('',#25581,#18294,#18295);
#15874=AXIS2_PLACEMENT_3D('',#25582,#18296,#18297);
#15875=AXIS2_PLACEMENT_3D('',#25583,#18298,#18299);
#15876=AXIS2_PLACEMENT_3D('',#25586,#18301,#18302);
#15877=AXIS2_PLACEMENT_3D('',#25587,#18303,#18304);
#15878=AXIS2_PLACEMENT_3D('',#25590,#18306,#18307);
#15879=AXIS2_PLACEMENT_3D('',#25591,#18308,#18309);
#15880=AXIS2_PLACEMENT_3D('',#25592,#18310,#18311);
#15881=AXIS2_PLACEMENT_3D('',#25595,#18313,#18314);
#15882=AXIS2_PLACEMENT_3D('',#25596,#18315,#18316);
#15883=AXIS2_PLACEMENT_3D('',#25599,#18318,#18319);
#15884=AXIS2_PLACEMENT_3D('',#25600,#18320,#18321);
#15885=AXIS2_PLACEMENT_3D('',#25601,#18322,#18323);
#15886=AXIS2_PLACEMENT_3D('',#25604,#18325,#18326);
#15887=AXIS2_PLACEMENT_3D('',#25605,#18327,#18328);
#15888=AXIS2_PLACEMENT_3D('',#25608,#18330,#18331);
#15889=AXIS2_PLACEMENT_3D('',#25609,#18332,#18333);
#15890=AXIS2_PLACEMENT_3D('',#25610,#18334,#18335);
#15891=AXIS2_PLACEMENT_3D('',#25613,#18337,#18338);
#15892=AXIS2_PLACEMENT_3D('',#25614,#18339,#18340);
#15893=AXIS2_PLACEMENT_3D('',#25617,#18342,#18343);
#15894=AXIS2_PLACEMENT_3D('',#25618,#18344,#18345);
#15895=AXIS2_PLACEMENT_3D('',#25619,#18346,#18347);
#15896=AXIS2_PLACEMENT_3D('',#25622,#18349,#18350);
#15897=AXIS2_PLACEMENT_3D('',#25623,#18351,#18352);
#15898=AXIS2_PLACEMENT_3D('',#25626,#18354,#18355);
#15899=AXIS2_PLACEMENT_3D('',#25627,#18356,#18357);
#15900=AXIS2_PLACEMENT_3D('',#25628,#18358,#18359);
#18172=DIRECTION('axis',(0.,0.,1.));
#18173=DIRECTION('refdir',(1.,0.,0.));
#18174=DIRECTION('center_axis',(1.,0.,-7.24866760671198E-15));
#18175=DIRECTION('ref_axis',(0.,-1.,-3.09315763145967E-17));
#18176=DIRECTION('center_axis',(-1.,0.,0.));
#18177=DIRECTION('ref_axis',(0.,-1.,-6.12323399573677E-17));
#18178=DIRECTION('center_axis',(-1.,0.,0.));
#18179=DIRECTION('ref_axis',(0.,-1.,-6.12323399573677E-17));
#18180=DIRECTION('',(-0.38268343236509,-0.923879532511287,2.63222533831604E-15));
#18181=DIRECTION('center_axis',(1.,0.,0.));
#18182=DIRECTION('ref_axis',(0.,-1.,0.));
#18183=DIRECTION('center_axis',(-1.,0.,0.));
#18184=DIRECTION('ref_axis',(0.,0.,1.));
#18185=DIRECTION('center_axis',(1.,0.,0.));
#18186=DIRECTION('ref_axis',(0.,0.,-1.));
#18187=DIRECTION('center_axis',(1.,0.,0.));
#18188=DIRECTION('ref_axis',(0.,0.78183148246803,-0.623489801858733));
#18189=DIRECTION('center_axis',(1.,0.,0.));
#18190=DIRECTION('ref_axis',(0.,0.974927912181824,0.222520933956314));
#18191=DIRECTION('center_axis',(1.,0.,0.));
#18192=DIRECTION('ref_axis',(0.,0.433883739117558,0.900968867902419));
#18193=DIRECTION('center_axis',(1.,0.,0.));
#18194=DIRECTION('ref_axis',(0.,-0.433883739117558,0.900968867902419));
#18195=DIRECTION('center_axis',(1.,0.,0.));
#18196=DIRECTION('ref_axis',(0.,-0.974927912181824,0.222520933956315));
#18197=DIRECTION('center_axis',(1.,0.,0.));
#18198=DIRECTION('ref_axis',(0.,-0.78183148246803,-0.623489801858733));
#18199=DIRECTION('',(0.,0.,1.));
#18200=DIRECTION('center_axis',(1.,0.,0.));
#18201=DIRECTION('ref_axis',(0.,0.,-1.));
#18202=DIRECTION('',(0.,0.,-1.));
#18203=DIRECTION('',(0.,1.,0.));
#18204=DIRECTION('center_axis',(1.,0.,0.));
#18205=DIRECTION('ref_axis',(0.,1.,0.));
#18206=DIRECTION('center_axis',(1.,0.,0.));
#18207=DIRECTION('ref_axis',(0.,0.,-1.));
#18208=DIRECTION('',(-0.707106781186548,0.707106781186548,8.65956056235493E-17));
#18209=DIRECTION('center_axis',(-0.707106781186555,0.70710678118654,0.));
#18210=DIRECTION('ref_axis',(0.,0.,1.));
#18211=DIRECTION('',(0.,0.,-1.));
#18212=DIRECTION('center_axis',(0.707106781186555,-0.70710678118654,0.));
#18213=DIRECTION('ref_axis',(0.70710678118654,0.707106781186555,0.));
#18214=DIRECTION('',(0.577350269189617,0.57735026918963,-0.57735026918963));
#18215=DIRECTION('center_axis',(-0.707106781186557,-0.707106781186538,0.));
#18216=DIRECTION('ref_axis',(0.,0.,1.));
#18217=DIRECTION('center_axis',(0.707106781186557,0.707106781186538,0.));
#18218=DIRECTION('ref_axis',(-0.707106781186538,0.707106781186557,0.));
#18219=DIRECTION('',(0.,0.,1.));
#18220=DIRECTION('',(-0.577350269189616,0.577350269189632,0.577350269189629));
#18221=DIRECTION('center_axis',(-0.707106781186543,0.,-0.707106781186552));
#18222=DIRECTION('ref_axis',(-0.707106781186552,0.,0.707106781186543));
#18223=DIRECTION('',(0.,-1.,0.));
#18224=DIRECTION('center_axis',(0.,-1.,0.));
#18225=DIRECTION('ref_axis',(1.,0.,0.));
#18226=DIRECTION('',(1.,0.,0.));
#18227=DIRECTION('',(0.,0.,1.));
#18228=DIRECTION('',(1.,0.,0.));
#18229=DIRECTION('center_axis',(0.,0.,1.));
#18230=DIRECTION('ref_axis',(1.,0.,0.));
#18231=DIRECTION('',(-1.,0.,0.));
#18232=DIRECTION('',(0.,1.,0.));
#18233=DIRECTION('center_axis',(1.,0.,0.));
#18234=DIRECTION('ref_axis',(0.,-1.83697019872103E-16,-1.));
#18235=DIRECTION('center_axis',(-0.707106781186555,-0.70710678118654,0.));
#18236=DIRECTION('ref_axis',(-0.70710678118654,0.707106781186555,0.));
#18237=DIRECTION('center_axis',(1.,0.,0.));
#18238=DIRECTION('ref_axis',(0.,0.,-1.));
#18239=DIRECTION('center_axis',(-0.70710678118653,0.707106781186565,0.));
#18240=DIRECTION('ref_axis',(0.707106781186565,0.70710678118653,0.));
#18241=DIRECTION('',(-1.,0.,0.));
#18242=DIRECTION('center_axis',(0.,1.,0.));
#18243=DIRECTION('ref_axis',(-1.,0.,0.));
#18244=DIRECTION('',(0.,0.,-1.));
#18245=DIRECTION('center_axis',(0.707106781186555,0.70710678118654,0.));
#18246=DIRECTION('ref_axis',(0.,0.,-1.));
#18247=DIRECTION('',(0.,0.,-1.));
#18248=DIRECTION('',(0.577350269189617,-0.57735026918963,0.57735026918963));
#18249=DIRECTION('center_axis',(0.70710678118653,-0.707106781186565,0.));
#18250=DIRECTION('ref_axis',(0.,0.,-1.));
#18251=DIRECTION('',(0.,0.,1.));
#18252=DIRECTION('',(-0.577350269189631,-0.577350269189623,-0.577350269189623));
#18253=DIRECTION('center_axis',(0.707106781186543,0.,-0.707106781186552));
#18254=DIRECTION('ref_axis',(-0.707106781186552,0.,-0.707106781186543));
#18255=DIRECTION('',(0.,-1.,0.));
#18256=DIRECTION('center_axis',(1.,0.,0.));
#18257=DIRECTION('ref_axis',(0.,0.,-1.));
#18258=DIRECTION('center_axis',(1.,0.,0.));
#18259=DIRECTION('ref_axis',(0.,0.,-1.));
#18260=DIRECTION('center_axis',(-1.,0.,0.));
#18261=DIRECTION('ref_axis',(0.,0.,-1.));
#18262=DIRECTION('center_axis',(-1.,0.,0.));
#18263=DIRECTION('ref_axis',(0.,0.78183148246803,-0.623489801858734));
#18264=DIRECTION('center_axis',(-1.,0.,0.));
#18265=DIRECTION('ref_axis',(0.,0.974927912181824,0.222520933956314));
#18266=DIRECTION('center_axis',(-1.,0.,0.));
#18267=DIRECTION('ref_axis',(0.,0.433883739117558,0.900968867902419));
#18268=DIRECTION('center_axis',(-1.,0.,0.));
#18269=DIRECTION('ref_axis',(0.,-0.433883739117558,0.900968867902419));
#18270=DIRECTION('center_axis',(-1.,0.,0.));
#18271=DIRECTION('ref_axis',(0.,-0.974927912181824,0.222520933956315));
#18272=DIRECTION('center_axis',(-1.,0.,0.));
#18273=DIRECTION('ref_axis',(0.,-0.78183148246803,-0.623489801858733));
#18274=DIRECTION('center_axis',(-1.,0.,0.));
#18275=DIRECTION('ref_axis',(0.,-0.78183148246803,-0.623489801858733));
#18276=DIRECTION('',(-1.,0.,0.));
#18277=DIRECTION('center_axis',(1.,0.,0.));
#18278=DIRECTION('ref_axis',(0.,-0.78183148246803,-0.623489801858733));
#18279=DIRECTION('center_axis',(1.,0.,0.));
#18280=DIRECTION('ref_axis',(0.,-0.78183148246803,-0.623489801858733));
#18281=DIRECTION('',(1.,0.,0.));
#18282=DIRECTION('center_axis',(1.,0.,0.));
#18283=DIRECTION('ref_axis',(0.,-0.78183148246803,-0.623489801858733));
#18284=DIRECTION('center_axis',(1.,0.,0.));
#18285=DIRECTION('ref_axis',(0.,-0.78183148246803,-0.623489801858733));
#18286=DIRECTION('center_axis',(-1.,0.,0.));
#18287=DIRECTION('ref_axis',(0.,-0.974927912181824,0.222520933956315));
#18288=DIRECTION('',(-1.,0.,0.));
#18289=DIRECTION('center_axis',(1.,0.,0.));
#18290=DIRECTION('ref_axis',(0.,-0.974927912181824,0.222520933956315));
#18291=DIRECTION('center_axis',(1.,0.,0.));
#18292=DIRECTION('ref_axis',(0.,-0.974927912181824,0.222520933956315));
#18293=DIRECTION('',(1.,0.,0.));
#18294=DIRECTION('center_axis',(1.,0.,0.));
#18295=DIRECTION('ref_axis',(0.,-0.974927912181824,0.222520933956315));
#18296=DIRECTION('center_axis',(1.,0.,0.));
#18297=DIRECTION('ref_axis',(0.,-0.974927912181824,0.222520933956315));
#18298=DIRECTION('center_axis',(-1.,0.,0.));
#18299=DIRECTION('ref_axis',(0.,-0.433883739117558,0.900968867902419));
#18300=DIRECTION('',(-1.,0.,0.));
#18301=DIRECTION('center_axis',(1.,0.,0.));
#18302=DIRECTION('ref_axis',(0.,-0.433883739117558,0.900968867902419));
#18303=DIRECTION('center_axis',(1.,0.,0.));
#18304=DIRECTION('ref_axis',(0.,-0.433883739117558,0.900968867902419));
#18305=DIRECTION('',(1.,0.,0.));
#18306=DIRECTION('center_axis',(1.,0.,0.));
#18307=DIRECTION('ref_axis',(0.,-0.433883739117558,0.900968867902419));
#18308=DIRECTION('center_axis',(1.,0.,0.));
#18309=DIRECTION('ref_axis',(0.,-0.433883739117558,0.900968867902419));
#18310=DIRECTION('center_axis',(-1.,0.,0.));
#18311=DIRECTION('ref_axis',(0.,0.433883739117558,0.900968867902419));
#18312=DIRECTION('',(-1.,0.,0.));
#18313=DIRECTION('center_axis',(1.,0.,0.));
#18314=DIRECTION('ref_axis',(0.,0.433883739117558,0.900968867902419));
#18315=DIRECTION('center_axis',(1.,0.,0.));
#18316=DIRECTION('ref_axis',(0.,0.433883739117558,0.900968867902419));
#18317=DIRECTION('',(1.,0.,0.));
#18318=DIRECTION('center_axis',(1.,0.,0.));
#18319=DIRECTION('ref_axis',(0.,0.433883739117558,0.900968867902419));
#18320=DIRECTION('center_axis',(1.,0.,0.));
#18321=DIRECTION('ref_axis',(0.,0.433883739117558,0.900968867902419));
#18322=DIRECTION('center_axis',(-1.,0.,0.));
#18323=DIRECTION('ref_axis',(0.,0.974927912181824,0.222520933956314));
#18324=DIRECTION('',(-1.,0.,0.));
#18325=DIRECTION('center_axis',(1.,0.,0.));
#18326=DIRECTION('ref_axis',(0.,0.974927912181824,0.222520933956314));
#18327=DIRECTION('center_axis',(1.,0.,0.));
#18328=DIRECTION('ref_axis',(0.,0.974927912181824,0.222520933956314));
#18329=DIRECTION('',(1.,0.,0.));
#18330=DIRECTION('center_axis',(1.,0.,0.));
#18331=DIRECTION('ref_axis',(0.,0.974927912181824,0.222520933956314));
#18332=DIRECTION('center_axis',(1.,0.,0.));
#18333=DIRECTION('ref_axis',(0.,0.974927912181824,0.222520933956314));
#18334=DIRECTION('center_axis',(-1.,0.,0.));
#18335=DIRECTION('ref_axis',(0.,0.78183148246803,-0.623489801858734));
#18336=DIRECTION('',(-1.,0.,0.));
#18337=DIRECTION('center_axis',(1.,0.,0.));
#18338=DIRECTION('ref_axis',(0.,0.78183148246803,-0.623489801858734));
#18339=DIRECTION('center_axis',(1.,0.,0.));
#18340=DIRECTION('ref_axis',(0.,0.78183148246803,-0.623489801858733));
#18341=DIRECTION('',(1.,0.,0.));
#18342=DIRECTION('center_axis',(1.,0.,0.));
#18343=DIRECTION('ref_axis',(0.,0.78183148246803,-0.623489801858733));
#18344=DIRECTION('center_axis',(1.,0.,0.));
#18345=DIRECTION('ref_axis',(0.,0.78183148246803,-0.623489801858734));
#18346=DIRECTION('center_axis',(-1.,0.,0.));
#18347=DIRECTION('ref_axis',(0.,0.,-1.));
#18348=DIRECTION('',(-1.,0.,0.));
#18349=DIRECTION('center_axis',(1.,0.,0.));
#18350=DIRECTION('ref_axis',(0.,0.,-1.));
#18351=DIRECTION('center_axis',(1.,0.,0.));
#18352=DIRECTION('ref_axis',(0.,0.,-1.));
#18353=DIRECTION('',(1.,0.,0.));
#18354=DIRECTION('center_axis',(1.,0.,0.));
#18355=DIRECTION('ref_axis',(0.,0.,-1.));
#18356=DIRECTION('center_axis',(1.,0.,0.));
#18357=DIRECTION('ref_axis',(0.,0.,-1.));
#18358=DIRECTION('center_axis',(1.,0.,0.));
#18359=DIRECTION('ref_axis',(0.,1.,0.));
#18360=DIRECTION('',(-1.,0.,0.));
#25468=CARTESIAN_POINT('',(0.,0.,0.));
#25469=CARTESIAN_POINT('Origin',(65.9767766952966,0.,-1.28139550481832E-15));
#25470=CARTESIAN_POINT('',(66.1535533905933,41.8535533905933,-5.12558201927329E-15));
#25471=CARTESIAN_POINT('',(66.1535533905933,-41.8535533905933,-5.12558201927329E-15));
#25472=CARTESIAN_POINT('Origin',(66.1535533905933,0.,-2.56279100963665E-15));
#25473=CARTESIAN_POINT('Origin',(66.1535533905933,0.,-2.56279100963665E-15));
#25474=CARTESIAN_POINT('',(65.8,41.,5.02105187650415E-15));
#25475=CARTESIAN_POINT('',(65.9767766952966,41.4267766952966,5.07331694788872E-15));
#25476=CARTESIAN_POINT('Origin',(65.8,0.,0.));
#25477=CARTESIAN_POINT('Origin',(65.8,41.5,0.));
#25478=CARTESIAN_POINT('',(65.8,-1.0421744260744E-15,36.51));
#25479=CARTESIAN_POINT('Origin',(65.8,0.,28.));
#25480=CARTESIAN_POINT('',(65.8,-28.5446674249078,22.7636126658624));
#25481=CARTESIAN_POINT('Origin',(65.8,-21.8912815091048,17.4577144520445));
#25482=CARTESIAN_POINT('',(65.8,-35.5946180737584,-8.12423929874504));
#25483=CARTESIAN_POINT('Origin',(65.8,-27.2979815410911,-6.2305861507768));
#25484=CARTESIAN_POINT('',(65.8,-15.8410953151821,-32.8943733671173));
#25485=CARTESIAN_POINT('Origin',(65.8,-12.1487446952916,-25.2271283012677));
#25486=CARTESIAN_POINT('',(65.8,15.841095315182,-32.8943733671173));
#25487=CARTESIAN_POINT('Origin',(65.8,12.1487446952916,-25.2271283012677));
#25488=CARTESIAN_POINT('',(65.8,35.5946180737584,-8.12423929874504));
#25489=CARTESIAN_POINT('Origin',(65.8,27.2979815410911,-6.23058615077681));
#25490=CARTESIAN_POINT('',(65.8,28.5446674249078,22.7636126658624));
#25491=CARTESIAN_POINT('Origin',(65.8,21.8912815091048,17.4577144520445));
#25492=CARTESIAN_POINT('',(65.8,-3.525,12.0031027238794));
#25493=CARTESIAN_POINT('',(65.8,-3.525,16.1));
#25494=CARTESIAN_POINT('',(65.8,-3.525,6.));
#25495=CARTESIAN_POINT('',(65.8,3.525,12.0031027238794));
#25496=CARTESIAN_POINT('Origin',(65.8,0.,0.));
#25497=CARTESIAN_POINT('',(65.8,3.525,16.1));
#25498=CARTESIAN_POINT('',(65.8,3.525,6.));
#25499=CARTESIAN_POINT('',(65.8,20.75,16.1));
#25500=CARTESIAN_POINT('Origin',(66.3,0.,0.));
#25501=CARTESIAN_POINT('',(66.8,-42.5,-5.20474889637625E-15));
#25502=CARTESIAN_POINT('Origin',(66.8,0.,0.));
#25503=CARTESIAN_POINT('',(66.3,-42.,-5.14351655641888E-15));
#25504=CARTESIAN_POINT('Origin',(66.05,-3.275,6.));
#25505=CARTESIAN_POINT('',(66.3,-3.025,15.6));
#25506=CARTESIAN_POINT('',(66.3,-3.025,12.1387592034771));
#25507=CARTESIAN_POINT('',(66.3,-3.025,6.));
#25508=CARTESIAN_POINT('Origin',(69.3249999999999,0.,0.));
#25509=CARTESIAN_POINT('',(65.8,-3.525,16.1));
#25510=CARTESIAN_POINT('Origin',(66.05,3.275,6.));
#25511=CARTESIAN_POINT('',(66.3,3.025,12.1387592034771));
#25512=CARTESIAN_POINT('Origin',(69.3249999999999,0.,0.));
#25513=CARTESIAN_POINT('',(66.3,3.025,15.6));
#25514=CARTESIAN_POINT('',(66.3,3.025,6.));
#25515=CARTESIAN_POINT('',(66.3,3.025,15.6));
#25516=CARTESIAN_POINT('Origin',(66.05,20.75,15.85));
#25517=CARTESIAN_POINT('',(66.3,20.75,15.6));
#25518=CARTESIAN_POINT('Origin',(65.7,-3.025,12.));
#25519=CARTESIAN_POINT('',(125.3,-3.025,15.6));
#25520=CARTESIAN_POINT('',(65.7,-3.025,15.6));
#25521=CARTESIAN_POINT('',(125.3,-3.025,12.1387592034771));
#25522=CARTESIAN_POINT('',(125.3,-3.025,6.));
#25523=CARTESIAN_POINT('',(95.8,-3.025,12.1387592034771));
#25524=CARTESIAN_POINT('Origin',(95.8,0.,15.6));
#25525=CARTESIAN_POINT('',(125.3,3.025,15.6));
#25526=CARTESIAN_POINT('',(125.9,3.025,15.6));
#25527=CARTESIAN_POINT('',(125.3,6.255,15.6));
#25528=CARTESIAN_POINT('Origin',(95.8,0.,0.));
#25529=CARTESIAN_POINT('',(125.8,-3.525,12.0031027238794));
#25530=CARTESIAN_POINT('Origin',(122.275,0.,0.));
#25531=CARTESIAN_POINT('',(125.8,3.525,12.0031027238794));
#25532=CARTESIAN_POINT('Origin',(125.8,0.,0.));
#25533=CARTESIAN_POINT('',(125.3,3.025,12.1387592034771));
#25534=CARTESIAN_POINT('Origin',(122.275,0.,0.));
#25535=CARTESIAN_POINT('',(95.8,3.025,12.1387592034771));
#25536=CARTESIAN_POINT('Origin',(125.9,3.025,12.));
#25537=CARTESIAN_POINT('',(125.3,3.025,6.));
#25538=CARTESIAN_POINT('Origin',(125.55,-3.275,6.));
#25539=CARTESIAN_POINT('',(125.8,-3.525,16.1));
#25540=CARTESIAN_POINT('',(125.8,-3.525,6.));
#25541=CARTESIAN_POINT('',(125.3,-3.025,15.6));
#25542=CARTESIAN_POINT('Origin',(125.55,3.275,6.));
#25543=CARTESIAN_POINT('',(125.8,3.525,16.1));
#25544=CARTESIAN_POINT('',(125.8,3.525,6.));
#25545=CARTESIAN_POINT('',(125.8,3.525,16.1));
#25546=CARTESIAN_POINT('Origin',(125.55,6.255,15.85));
#25547=CARTESIAN_POINT('',(125.8,6.255,16.1));
#25548=CARTESIAN_POINT('Origin',(125.8,12.51,0.));
#25549=CARTESIAN_POINT('',(125.8,-42.5,-5.20474889637625E-15));
#25550=CARTESIAN_POINT('Origin',(125.8,0.,0.));
#25551=CARTESIAN_POINT('',(125.8,-6.12323399573677E-16,33.));
#25552=CARTESIAN_POINT('Origin',(125.8,0.,28.));
#25553=CARTESIAN_POINT('',(125.8,-25.800438921445,20.5751634613382));
#25554=CARTESIAN_POINT('Origin',(125.8,-21.8912815091048,17.4577144520445));
#25555=CARTESIAN_POINT('',(125.8,-32.1726211020002,-7.34319082055837));
#25556=CARTESIAN_POINT('Origin',(125.8,-27.2979815410911,-6.2305861507768));
#25557=CARTESIAN_POINT('',(125.8,-14.3181633908794,-29.7319726407798));
#25558=CARTESIAN_POINT('Origin',(125.8,-12.1487446952916,-25.2271283012677));
#25559=CARTESIAN_POINT('',(125.8,14.3181633908794,-29.7319726407798));
#25560=CARTESIAN_POINT('Origin',(125.8,12.1487446952916,-25.2271283012677));
#25561=CARTESIAN_POINT('',(125.8,32.1726211020002,-7.34319082055838));
#25562=CARTESIAN_POINT('Origin',(125.8,27.2979815410911,-6.23058615077681));
#25563=CARTESIAN_POINT('',(125.8,25.800438921445,20.5751634613382));
#25564=CARTESIAN_POINT('Origin',(125.8,21.8912815091048,17.4577144520445));
#25565=CARTESIAN_POINT('Origin',(125.8,21.8912815091048,17.4577144520445));
#25566=CARTESIAN_POINT('',(119.,25.800438921445,20.5751634613382));
#25567=CARTESIAN_POINT('',(125.8,25.800438921445,20.5751634613382));
#25568=CARTESIAN_POINT('Origin',(119.,21.8912815091048,17.4577144520445));
#25569=CARTESIAN_POINT('Origin',(65.8,21.8912815091048,17.4577144520445));
#25570=CARTESIAN_POINT('',(119.,28.5446674249078,22.7636126658624));
#25571=CARTESIAN_POINT('',(65.8,28.5446674249078,22.7636126658624));
#25572=CARTESIAN_POINT('Origin',(119.,21.8912815091048,17.4577144520445));
#25573=CARTESIAN_POINT('Origin',(119.,21.8912815091048,17.4577144520445));
#25574=CARTESIAN_POINT('Origin',(125.8,27.2979815410911,-6.23058615077681));
#25575=CARTESIAN_POINT('',(119.,32.1726211020002,-7.34319082055838));
#25576=CARTESIAN_POINT('',(125.8,32.1726211020002,-7.34319082055838));
#25577=CARTESIAN_POINT('Origin',(119.,27.2979815410911,-6.23058615077681));
#25578=CARTESIAN_POINT('Origin',(65.8,27.2979815410911,-6.23058615077681));
#25579=CARTESIAN_POINT('',(119.,35.5946180737584,-8.12423929874504));
#25580=CARTESIAN_POINT('',(65.8,35.5946180737584,-8.12423929874504));
#25581=CARTESIAN_POINT('Origin',(119.,27.2979815410911,-6.23058615077681));
#25582=CARTESIAN_POINT('Origin',(119.,27.2979815410911,-6.23058615077681));
#25583=CARTESIAN_POINT('Origin',(125.8,12.1487446952916,-25.2271283012677));
#25584=CARTESIAN_POINT('',(119.,14.3181633908794,-29.7319726407798));
#25585=CARTESIAN_POINT('',(125.8,14.3181633908794,-29.7319726407798));
#25586=CARTESIAN_POINT('Origin',(119.,12.1487446952916,-25.2271283012677));
#25587=CARTESIAN_POINT('Origin',(65.8,12.1487446952916,-25.2271283012677));
#25588=CARTESIAN_POINT('',(119.,15.841095315182,-32.8943733671173));
#25589=CARTESIAN_POINT('',(65.8,15.841095315182,-32.8943733671173));
#25590=CARTESIAN_POINT('Origin',(119.,12.1487446952916,-25.2271283012677));
#25591=CARTESIAN_POINT('Origin',(119.,12.1487446952916,-25.2271283012677));
#25592=CARTESIAN_POINT('Origin',(125.8,-12.1487446952916,-25.2271283012677));
#25593=CARTESIAN_POINT('',(119.,-14.3181633908794,-29.7319726407798));
#25594=CARTESIAN_POINT('',(125.8,-14.3181633908794,-29.7319726407798));
#25595=CARTESIAN_POINT('Origin',(119.,-12.1487446952916,-25.2271283012677));
#25596=CARTESIAN_POINT('Origin',(65.8,-12.1487446952916,-25.2271283012677));
#25597=CARTESIAN_POINT('',(119.,-15.8410953151821,-32.8943733671173));
#25598=CARTESIAN_POINT('',(65.8,-15.8410953151821,-32.8943733671173));
#25599=CARTESIAN_POINT('Origin',(119.,-12.1487446952916,-25.2271283012677));
#25600=CARTESIAN_POINT('Origin',(119.,-12.1487446952916,-25.2271283012677));
#25601=CARTESIAN_POINT('Origin',(125.8,-27.2979815410911,-6.2305861507768));
#25602=CARTESIAN_POINT('',(119.,-32.1726211020002,-7.34319082055837));
#25603=CARTESIAN_POINT('',(125.8,-32.1726211020002,-7.34319082055837));
#25604=CARTESIAN_POINT('Origin',(119.,-27.2979815410911,-6.2305861507768));
#25605=CARTESIAN_POINT('Origin',(65.8,-27.2979815410911,-6.2305861507768));
#25606=CARTESIAN_POINT('',(119.,-35.5946180737584,-8.12423929874504));
#25607=CARTESIAN_POINT('',(65.8,-35.5946180737584,-8.12423929874504));
#25608=CARTESIAN_POINT('Origin',(119.,-27.2979815410911,-6.2305861507768));
#25609=CARTESIAN_POINT('Origin',(119.,-27.2979815410911,-6.2305861507768));
#25610=CARTESIAN_POINT('Origin',(125.8,-21.8912815091048,17.4577144520445));
#25611=CARTESIAN_POINT('',(119.,-25.800438921445,20.5751634613382));
#25612=CARTESIAN_POINT('',(125.8,-25.800438921445,20.5751634613382));
#25613=CARTESIAN_POINT('Origin',(119.,-21.8912815091048,17.4577144520445));
#25614=CARTESIAN_POINT('Origin',(65.8,-21.8912815091048,17.4577144520445));
#25615=CARTESIAN_POINT('',(119.,-28.5446674249078,22.7636126658624));
#25616=CARTESIAN_POINT('',(65.8,-28.5446674249078,22.7636126658624));
#25617=CARTESIAN_POINT('Origin',(119.,-21.8912815091048,17.4577144520445));
#25618=CARTESIAN_POINT('Origin',(119.,-21.8912815091048,17.4577144520445));
#25619=CARTESIAN_POINT('Origin',(125.8,0.,28.));
#25620=CARTESIAN_POINT('',(119.,-6.12323399573677E-16,33.));
#25621=CARTESIAN_POINT('',(125.8,6.12323399573677E-16,33.));
#25622=CARTESIAN_POINT('Origin',(119.,0.,28.));
#25623=CARTESIAN_POINT('Origin',(65.8,0.,28.));
#25624=CARTESIAN_POINT('',(119.,-1.0421744260744E-15,36.51));
#25625=CARTESIAN_POINT('',(65.8,-1.0421744260744E-15,36.51));
#25626=CARTESIAN_POINT('Origin',(119.,0.,28.));
#25627=CARTESIAN_POINT('Origin',(119.,0.,28.));
#25628=CARTESIAN_POINT('Origin',(96.3,0.,0.));
#25629=CARTESIAN_POINT('',(96.3,-42.5,-5.20474889637625E-15));
#38478=UNCERTAINTY_MEASURE_WITH_UNIT(LENGTH_MEASURE(0.01),#38508,
'DISTANCE_ACCURACY_VALUE',
'Maximum model space distance between geometric entities at asserted c
onnectivities');
#38490=UNCERTAINTY_MEASURE_WITH_UNIT(LENGTH_MEASURE(0.01),#38508,
'DISTANCE_ACCURACY_VALUE',
'Maximum model space distance between geometric entities at asserted c
onnectivities');
#38495=(
GEOMETRIC_REPRESENTATION_CONTEXT(3)
GLOBAL_UNCERTAINTY_ASSIGNED_CONTEXT((#38478))
GLOBAL_UNIT_ASSIGNED_CONTEXT((#38508,#38510,#38511))
REPRESENTATION_CONTEXT('','3D')
);
#38507=(
GEOMETRIC_REPRESENTATION_CONTEXT(3)
GLOBAL_UNCERTAINTY_ASSIGNED_CONTEXT((#38490))
GLOBAL_UNIT_ASSIGNED_CONTEXT((#38508,#38510,#38511))
REPRESENTATION_CONTEXT('','3D')
);
#38508=(
LENGTH_UNIT()
NAMED_UNIT(*)
SI_UNIT(.MILLI.,.METRE.)
);
#38510=(
NAMED_UNIT(*)
PLANE_ANGLE_UNIT()
SI_UNIT($,.RADIAN.)
);
#38511=(
NAMED_UNIT(*)
SI_UNIT($,.STERADIAN.)
SOLID_ANGLE_UNIT()
);
#38516=SHAPE_DEFINITION_REPRESENTATION(#38532,#38578);
#38532=PRODUCT_DEFINITION_SHAPE('',$,#38595);
#38578=SHAPE_REPRESENTATION('',(#15825),#38495);
#38590=PRODUCT_DEFINITION_CONTEXT('part definition',#38640,'design');
#38595=PRODUCT_DEFINITION('2026-10-26-01-10-46-823',
'04_Cylinder_Barrel',#38611,#38590);
#38611=PRODUCT_DEFINITION_FORMATION('',$,#38646);
#38640=APPLICATION_CONTEXT(
'Core Data for Automotive Mechanical Design Process');
#38641=PRODUCT_CONTEXT('part definition',#38640,'mechanical');
#38646=PRODUCT('2026-10-26-01-10-46-823','04_Cylinder_Barrel',$,(#38641));
#38728=COLOUR_RGB('Off White',0.89,0.88,0.83);
#38729=FILL_AREA_STYLE_COLOUR('',#38728);
#38730=FILL_AREA_STYLE('',(#38729));
#38731=SURFACE_STYLE_FILL_AREA(#38730);
#38732=SURFACE_SIDE_STYLE('',(#38731));
#38733=SURFACE_STYLE_USAGE(.BOTH.,#38732);
#38734=PRESENTATION_STYLE_ASSIGNMENT((#38733));
ENDSEC;
END-ISO-10303-21;
